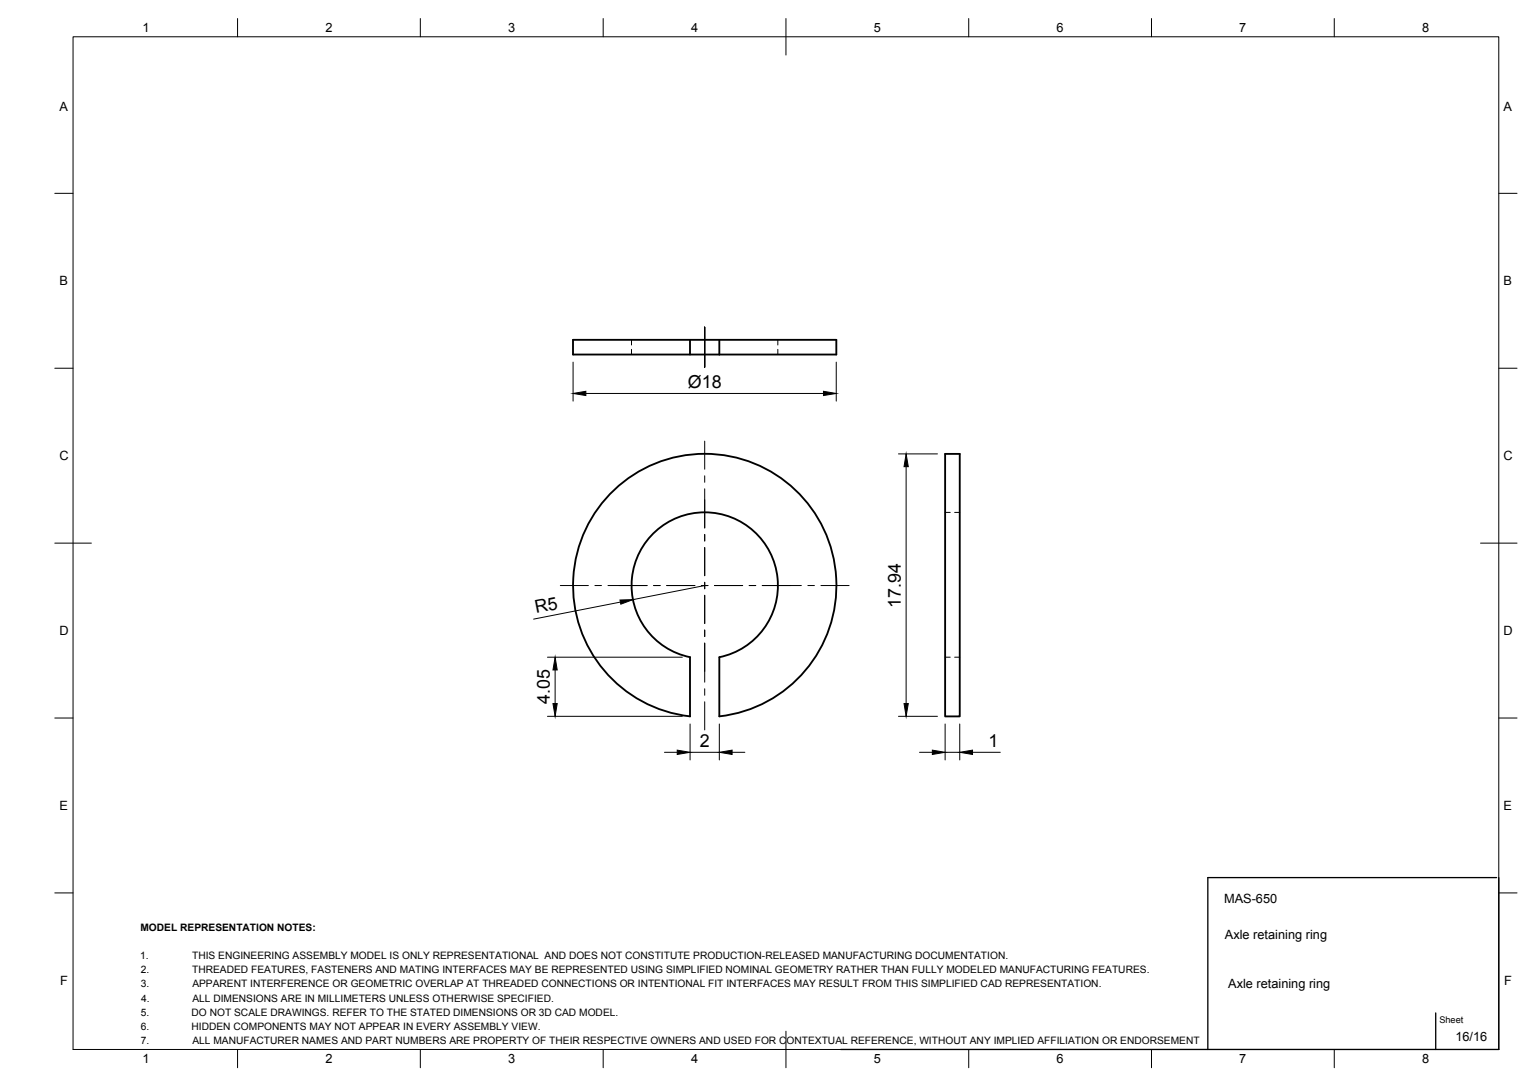
ISO-10303-21;
HEADER;
/* Generated by software containing ST-Developer
 * from STEP Tools, Inc. (www.steptools.com) 
 */

FILE_DESCRIPTION(
/* description */ ('Independent manual traversing gantry with native reusable aluminum pr
ofiles,180mm captured carriage travel, four bronze-bushed rollers, lin
ked ideal rolling motion, bonded acetal lateral guides, positive welde
d end stops and fully retained axle stacks. Editable native profile cu
t lengths220/400mm. Tool attachments viaM6 bridge-plate taps; mounted 
tool outside assembly. Welds, anchors, adhesives, fits, traction, load
/speed/structural/life ratings unassigned.'),
/* implementation_level */ '2;1');

FILE_NAME(
/* name */ 'Axle retaining ring.step',
/* time_stamp */ '2026-11-09T20:04:38-08:00',
/* author */ (''),
/* organization */ (''),
/* preprocessor_version */ 'ST-DEVELOPER v20.2',
/* originating_system */ 'Autodesk Translation Framework v15.17.0.0',
/* authorisation */ '');

FILE_SCHEMA (('AUTOMOTIVE_DESIGN { 1 0 10303 214 3 1 1 }'));
ENDSEC;

DATA;
#10=MECHANICAL_DESIGN_GEOMETRIC_PRESENTATION_REPRESENTATION('',(#483),#13231);
#451=SHAPE_REPRESENTATION_RELATIONSHIP('SRR','None',#13340,#467);
#467=ADVANCED_BREP_SHAPE_REPRESENTATION('',(#499),#13227);
#483=STYLED_ITEM('',(#13428),#499);
#499=MANIFOLD_SOLID_BREP('Body1',#4163);
#623=PLANE('',#4641);
#624=PLANE('',#4642);
#625=PLANE('',#4643);
#626=PLANE('',#4650);
#836=FACE_OUTER_BOUND('',#1100,.T.);
#837=FACE_OUTER_BOUND('',#1101,.T.);
#838=FACE_OUTER_BOUND('',#1102,.T.);
#839=FACE_OUTER_BOUND('',#1103,.T.);
#840=FACE_OUTER_BOUND('',#1104,.T.);
#841=FACE_OUTER_BOUND('',#1105,.T.);
#1100=EDGE_LOOP('',(#3738,#3739,#3740,#3741));
#1101=EDGE_LOOP('',(#3742,#3743,#3744,#3745));
#1102=EDGE_LOOP('',(#3746,#3747,#3748,#3749));
#1103=EDGE_LOOP('',(#3750,#3751,#3752,#3753));
#1104=EDGE_LOOP('',(#3754,#3755,#3756,#3757));
#1105=EDGE_LOOP('',(#3758,#3759,#3760,#3761));
#1372=LINE('',#13071,#1634);
#1373=LINE('',#13073,#1635);
#1374=LINE('',#13075,#1636);
#1375=LINE('',#13076,#1637);
#1376=LINE('',#13080,#1638);
#1377=LINE('',#13082,#1639);
#1378=LINE('',#13084,#1640);
#1379=LINE('',#13085,#1641);
#1634=VECTOR('',#5579,10.);
#1635=VECTOR('',#5580,10.);
#1636=VECTOR('',#5581,10.);
#1637=VECTOR('',#5582,10.);
#1638=VECTOR('',#5585,10.);
#1639=VECTOR('',#5586,10.);
#1640=VECTOR('',#5587,10.);
#1641=VECTOR('',#5588,10.);
#1736=CIRCLE('',#4644,9.);
#1737=CIRCLE('',#4645,5.);
#1738=CIRCLE('',#4647,5.);
#1739=CIRCLE('',#4649,9.);
#2104=VERTEX_POINT('',#13069);
#2105=VERTEX_POINT('',#13070);
#2106=VERTEX_POINT('',#13072);
#2107=VERTEX_POINT('',#13074);
#2108=VERTEX_POINT('',#13078);
#2109=VERTEX_POINT('',#13079);
#2110=VERTEX_POINT('',#13081);
#2111=VERTEX_POINT('',#13083);
#2652=EDGE_CURVE('',#2104,#2105,#1372,.T.);
#2653=EDGE_CURVE('',#2106,#2104,#1373,.T.);
#2654=EDGE_CURVE('',#2107,#2106,#1374,.T.);
#2655=EDGE_CURVE('',#2105,#2107,#1375,.T.);
#2656=EDGE_CURVE('',#2108,#2109,#1376,.T.);
#2657=EDGE_CURVE('',#2110,#2108,#1377,.T.);
#2658=EDGE_CURVE('',#2111,#2110,#1378,.T.);
#2659=EDGE_CURVE('',#2109,#2111,#1379,.T.);
#2660=EDGE_CURVE('',#2106,#2111,#1736,.T.);
#2661=EDGE_CURVE('',#2109,#2104,#1737,.T.);
#2662=EDGE_CURVE('',#2108,#2105,#1738,.T.);
#2663=EDGE_CURVE('',#2107,#2110,#1739,.T.);
#3738=ORIENTED_EDGE('',*,*,#2652,.F.);
#3739=ORIENTED_EDGE('',*,*,#2653,.F.);
#3740=ORIENTED_EDGE('',*,*,#2654,.F.);
#3741=ORIENTED_EDGE('',*,*,#2655,.F.);
#3742=ORIENTED_EDGE('',*,*,#2656,.F.);
#3743=ORIENTED_EDGE('',*,*,#2657,.F.);
#3744=ORIENTED_EDGE('',*,*,#2658,.F.);
#3745=ORIENTED_EDGE('',*,*,#2659,.F.);
#3746=ORIENTED_EDGE('',*,*,#2659,.T.);
#3747=ORIENTED_EDGE('',*,*,#2660,.F.);
#3748=ORIENTED_EDGE('',*,*,#2653,.T.);
#3749=ORIENTED_EDGE('',*,*,#2661,.F.);
#3750=ORIENTED_EDGE('',*,*,#2656,.T.);
#3751=ORIENTED_EDGE('',*,*,#2661,.T.);
#3752=ORIENTED_EDGE('',*,*,#2652,.T.);
#3753=ORIENTED_EDGE('',*,*,#2662,.F.);
#3754=ORIENTED_EDGE('',*,*,#2658,.T.);
#3755=ORIENTED_EDGE('',*,*,#2663,.F.);
#3756=ORIENTED_EDGE('',*,*,#2654,.T.);
#3757=ORIENTED_EDGE('',*,*,#2660,.T.);
#3758=ORIENTED_EDGE('',*,*,#2657,.T.);
#3759=ORIENTED_EDGE('',*,*,#2662,.T.);
#3760=ORIENTED_EDGE('',*,*,#2655,.T.);
#3761=ORIENTED_EDGE('',*,*,#2663,.T.);
#3922=CYLINDRICAL_SURFACE('',#4646,5.);
#3923=CYLINDRICAL_SURFACE('',#4648,9.);
#4133=ADVANCED_FACE('',(#836),#623,.F.);
#4134=ADVANCED_FACE('',(#837),#624,.F.);
#4135=ADVANCED_FACE('',(#838),#625,.F.);
#4136=ADVANCED_FACE('',(#839),#3922,.F.);
#4137=ADVANCED_FACE('',(#840),#3923,.T.);
#4138=ADVANCED_FACE('',(#841),#626,.T.);
#4163=CLOSED_SHELL('',(#4133,#4134,#4135,#4136,#4137,#4138));
#4640=AXIS2_PLACEMENT_3D('',#13067,#5575,#5576);
#4641=AXIS2_PLACEMENT_3D('',#13068,#5577,#5578);
#4642=AXIS2_PLACEMENT_3D('',#13077,#5583,#5584);
#4643=AXIS2_PLACEMENT_3D('',#13086,#5589,#5590);
#4644=AXIS2_PLACEMENT_3D('',#13087,#5591,#5592);
#4645=AXIS2_PLACEMENT_3D('',#13088,#5593,#5594);
#4646=AXIS2_PLACEMENT_3D('',#13089,#5595,#5596);
#4647=AXIS2_PLACEMENT_3D('',#13090,#5597,#5598);
#4648=AXIS2_PLACEMENT_3D('',#13091,#5599,#5600);
#4649=AXIS2_PLACEMENT_3D('',#13092,#5601,#5602);
#4650=AXIS2_PLACEMENT_3D('',#13093,#5603,#5604);
#5575=DIRECTION('axis',(0.,0.,1.));
#5576=DIRECTION('refdir',(1.,0.,0.));
#5577=DIRECTION('center_axis',(-1.,0.,0.));
#5578=DIRECTION('ref_axis',(0.,1.,0.));
#5579=DIRECTION('',(0.,0.,1.));
#5580=DIRECTION('',(0.,-1.,0.));
#5581=DIRECTION('',(0.,0.,-1.));
#5582=DIRECTION('',(0.,1.,0.));
#5583=DIRECTION('center_axis',(1.,0.,0.));
#5584=DIRECTION('ref_axis',(0.,-1.,0.));
#5585=DIRECTION('',(0.,0.,-1.));
#5586=DIRECTION('',(0.,-1.,0.));
#5587=DIRECTION('',(0.,0.,1.));
#5588=DIRECTION('',(0.,1.,0.));
#5589=DIRECTION('center_axis',(0.,0.,1.));
#5590=DIRECTION('ref_axis',(1.,0.,0.));
#5591=DIRECTION('center_axis',(0.,0.,1.));
#5592=DIRECTION('ref_axis',(1.,0.,0.));
#5593=DIRECTION('center_axis',(0.,0.,-1.));
#5594=DIRECTION('ref_axis',(1.,0.,0.));
#5595=DIRECTION('center_axis',(0.,0.,1.));
#5596=DIRECTION('ref_axis',(6.12323399573677E-17,-1.,0.));
#5597=DIRECTION('center_axis',(0.,0.,-1.));
#5598=DIRECTION('ref_axis',(1.,0.,0.));
#5599=DIRECTION('center_axis',(0.,0.,1.));
#5600=DIRECTION('ref_axis',(6.12323399573677E-17,-1.,0.));
#5601=DIRECTION('center_axis',(0.,0.,1.));
#5602=DIRECTION('ref_axis',(1.,0.,0.));
#5603=DIRECTION('center_axis',(0.,0.,1.));
#5604=DIRECTION('ref_axis',(1.,0.,0.));
#13067=CARTESIAN_POINT('',(0.,0.,0.));
#13068=CARTESIAN_POINT('Origin',(-1.,0.,1.));
#13069=CARTESIAN_POINT('',(-1.,4.89897948556636,0.));
#13070=CARTESIAN_POINT('',(-1.,4.89897948556636,1.));
#13071=CARTESIAN_POINT('',(-1.,4.89897948556636,0.));
#13072=CARTESIAN_POINT('',(-1.,8.94427190999916,0.));
#13073=CARTESIAN_POINT('',(-1.,0.,0.));
#13074=CARTESIAN_POINT('',(-1.,8.94427190999916,1.));
#13075=CARTESIAN_POINT('',(-1.,8.94427190999916,0.));
#13076=CARTESIAN_POINT('',(-1.,0.,1.));
#13077=CARTESIAN_POINT('Origin',(1.,18.,1.));
#13078=CARTESIAN_POINT('',(1.,4.89897948556636,1.));
#13079=CARTESIAN_POINT('',(1.,4.89897948556636,0.));
#13080=CARTESIAN_POINT('',(1.,4.89897948556636,0.));
#13081=CARTESIAN_POINT('',(1.,8.94427190999916,1.));
#13082=CARTESIAN_POINT('',(1.,9.,1.));
#13083=CARTESIAN_POINT('',(1.,8.94427190999916,0.));
#13084=CARTESIAN_POINT('',(1.,8.94427190999916,0.));
#13085=CARTESIAN_POINT('',(1.,9.,0.));
#13086=CARTESIAN_POINT('Origin',(0.,0.,0.));
#13087=CARTESIAN_POINT('Origin',(0.,0.,0.));
#13088=CARTESIAN_POINT('Origin',(0.,0.,0.));
#13089=CARTESIAN_POINT('Origin',(0.,0.,0.));
#13090=CARTESIAN_POINT('Origin',(0.,0.,1.));
#13091=CARTESIAN_POINT('Origin',(0.,0.,0.));
#13092=CARTESIAN_POINT('Origin',(0.,0.,1.));
#13093=CARTESIAN_POINT('Origin',(0.,0.,1.));
#13209=UNCERTAINTY_MEASURE_WITH_UNIT(LENGTH_MEASURE(0.01),#13232,
'DISTANCE_ACCURACY_VALUE',
'Maximum model space distance between geometric entities at asserted c
onnectivities');
#13213=UNCERTAINTY_MEASURE_WITH_UNIT(LENGTH_MEASURE(0.01),#13232,
'DISTANCE_ACCURACY_VALUE',
'Maximum model space distance between geometric entities at asserted c
onnectivities');
#13227=(
GEOMETRIC_REPRESENTATION_CONTEXT(3)
GLOBAL_UNCERTAINTY_ASSIGNED_CONTEXT((#13209))
GLOBAL_UNIT_ASSIGNED_CONTEXT((#13232,#13234,#13235))
REPRESENTATION_CONTEXT('','3D')
);
#13231=(
GEOMETRIC_REPRESENTATION_CONTEXT(3)
GLOBAL_UNCERTAINTY_ASSIGNED_CONTEXT((#13213))
GLOBAL_UNIT_ASSIGNED_CONTEXT((#13232,#13234,#13235))
REPRESENTATION_CONTEXT('','3D')
);
#13232=(
LENGTH_UNIT()
NAMED_UNIT(*)
SI_UNIT(.MILLI.,.METRE.)
);
#13234=(
NAMED_UNIT(*)
PLANE_ANGLE_UNIT()
SI_UNIT($,.RADIAN.)
);
#13235=(
NAMED_UNIT(*)
SI_UNIT($,.STERADIAN.)
SOLID_ANGLE_UNIT()
);
#13249=SHAPE_DEFINITION_REPRESENTATION(#13266,#13340);
#13266=PRODUCT_DEFINITION_SHAPE('',$,#13358);
#13340=SHAPE_REPRESENTATION('',(#4640),#13227);
#13344=PRODUCT_DEFINITION_CONTEXT('part definition',#13397,'design');
#13358=PRODUCT_DEFINITION('Axle retaining ring','Axle retaining ring',#13375,
#13344);
#13375=PRODUCT_DEFINITION_FORMATION('',$,#13412);
#13397=APPLICATION_CONTEXT(
'Core Data for Automotive Mechanical Design Process');
#13398=PRODUCT_CONTEXT('part definition',#13397,'mechanical');
#13412=PRODUCT('Axle retaining ring','Axle retaining ring',$,(#13398));
#13428=PRESENTATION_STYLE_ASSIGNMENT((#13442));
#13442=SURFACE_STYLE_USAGE(.BOTH.,#13456);
#13456=SURFACE_SIDE_STYLE('',(#13470));
#13470=SURFACE_STYLE_FILL_AREA(#13484);
#13484=FILL_AREA_STYLE('Dark gray',(#13498));
#13498=FILL_AREA_STYLE_COLOUR('Dark gray',#13512);
#13512=COLOUR_RGB('Dark gray',0.250980392156863,0.282352941176471,0.32156862745098);
ENDSEC;
END-ISO-10303-21;
